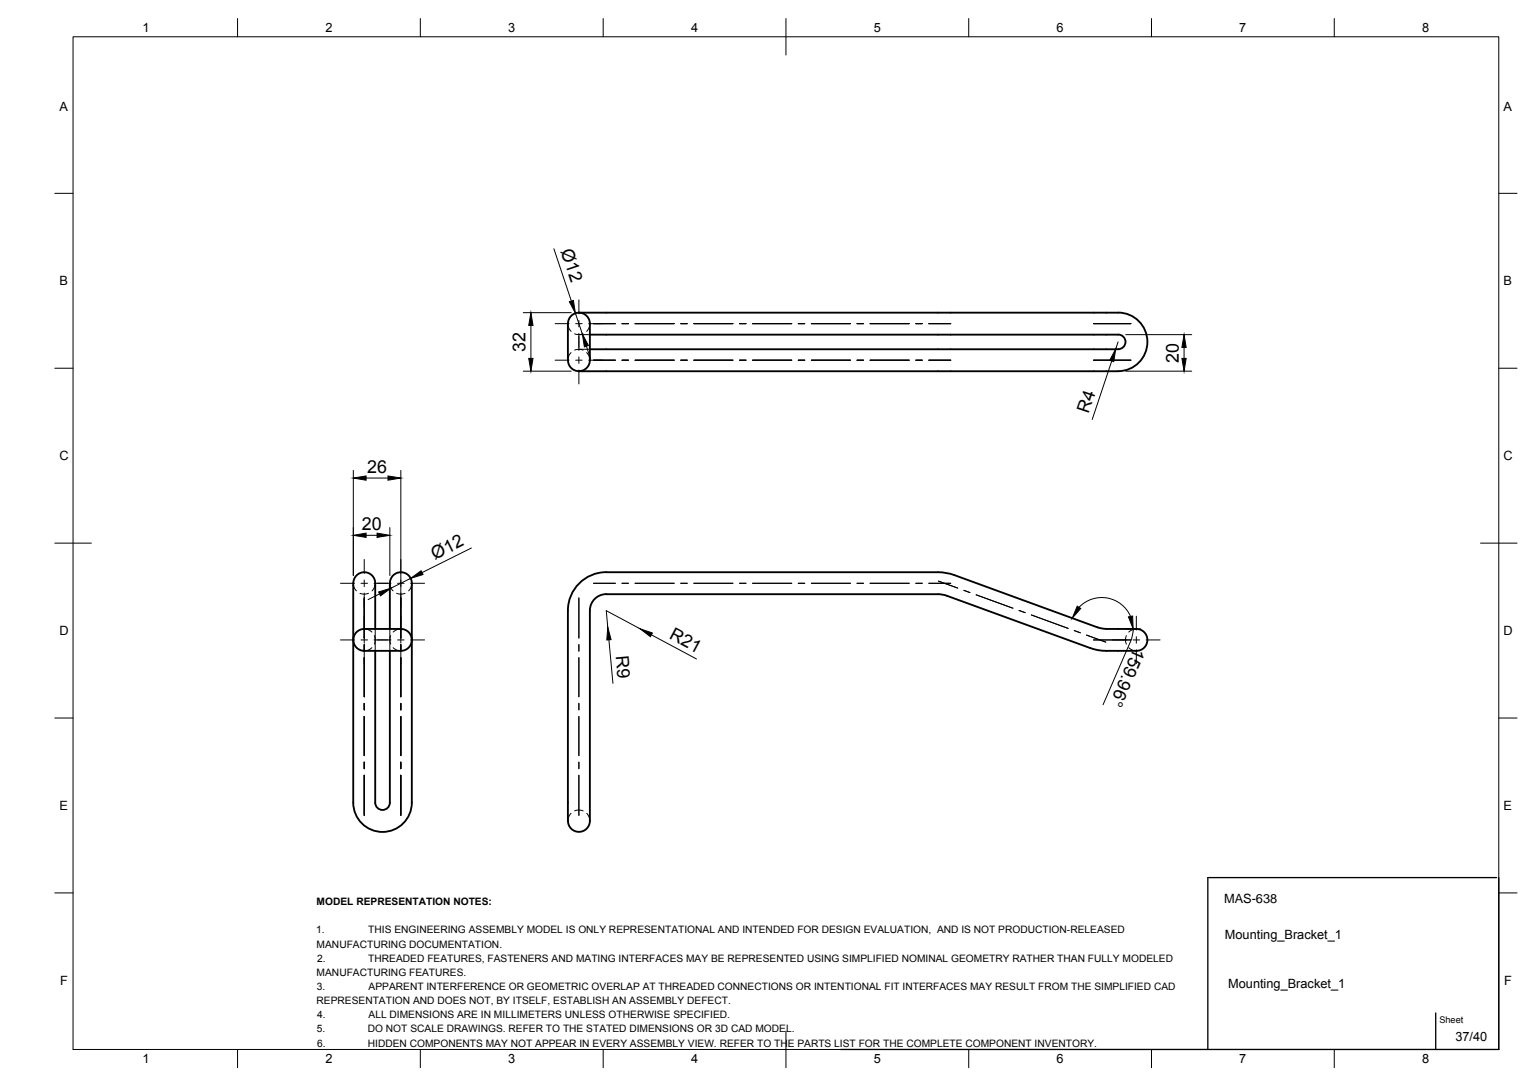
ISO-10303-21;
HEADER;
FILE_DESCRIPTION((''),'2;1');
FILE_NAME('Mounting_Bracket_1.step','2026-10-09T12:00:21-07:00',(''),(''),'','','');
FILE_SCHEMA (('AUTOMOTIVE_DESIGN { 1 0 10303 214 3 1 1 }'));
ENDSEC;
DATA;
#10=MECHANICAL_DESIGN_GEOMETRIC_PRESENTATION_REPRESENTATION('',(#432),#10334);
#160=CYLINDRICAL_SURFACE('',#4275,0.600000000000001) ;
#161=CYLINDRICAL_SURFACE('',#4276,0.600000000000001) ;
#162=CYLINDRICAL_SURFACE('',#4277,0.599999999999996) ;
#163=CYLINDRICAL_SURFACE('',#4278,0.600000000000001) ;
#164=CYLINDRICAL_SURFACE('',#4279,0.600000000000001) ;
#165=CYLINDRICAL_SURFACE('',#4280,0.600000000000001) ;
#166=CYLINDRICAL_SURFACE('',#4281,0.599999999999996) ;
#167=CYLINDRICAL_SURFACE('',#4282,0.600000000000001) ;
#360=SHAPE_REPRESENTATION_RELATIONSHIP('SRR','None',#10478,#392) ;
#392=ADVANCED_BREP_SHAPE_REPRESENTATION('',(#464),#10330) ;
#432=STYLED_ITEM('',(#10631),#464) ;
#464=MANIFOLD_SOLID_BREP('Body1',#3586) ;
#658=LINE('',#9983,#816) ;
#659=LINE('',#9985,#817) ;
#660=LINE('',#9987,#818) ;
#661=LINE('',#9989,#819) ;
#662=LINE('',#9991,#820) ;
#663=LINE('',#9993,#821) ;
#664=LINE('',#9995,#822) ;
#665=LINE('',#9997,#823) ;
#816=VECTOR('',#5236,0.600000000000001) ;
#817=VECTOR('',#5239,0.600000000000001) ;
#818=VECTOR('',#5242,0.599999999999996) ;
#819=VECTOR('',#5245,0.600000000000001) ;
#820=VECTOR('',#5248,0.600000000000001) ;
#821=VECTOR('',#5251,0.600000000000001) ;
#822=VECTOR('',#5254,0.599999999999996) ;
#823=VECTOR('',#5257,0.600000000000001) ;
#986=FACE_OUTER_BOUND('',#1194,.T.) ;
#987=FACE_OUTER_BOUND('',#1195,.T.) ;
#988=FACE_OUTER_BOUND('',#1196,.T.) ;
#989=FACE_OUTER_BOUND('',#1197,.T.) ;
#990=FACE_OUTER_BOUND('',#1198,.T.) ;
#991=FACE_OUTER_BOUND('',#1199,.T.) ;
#992=FACE_OUTER_BOUND('',#1200,.T.) ;
#993=FACE_OUTER_BOUND('',#1201,.T.) ;
#994=FACE_OUTER_BOUND('',#1202,.T.) ;
#995=FACE_OUTER_BOUND('',#1203,.T.) ;
#996=FACE_OUTER_BOUND('',#1204,.T.) ;
#997=FACE_OUTER_BOUND('',#1205,.T.) ;
#998=FACE_OUTER_BOUND('',#1206,.T.) ;
#999=FACE_OUTER_BOUND('',#1207,.T.) ;
#1000=FACE_OUTER_BOUND('',#1208,.T.) ;
#1001=FACE_OUTER_BOUND('',#1209,.T.) ;
#1194=EDGE_LOOP('',(#2965,#2966,#2967,#2968,#2969)) ;
#1195=EDGE_LOOP('',(#2970,#2971,#2972,#2973)) ;
#1196=EDGE_LOOP('',(#2974,#2975,#2976,#2977,#2978,#2979)) ;
#1197=EDGE_LOOP('',(#2980,#2981,#2982,#2983,#2984,#2985)) ;
#1198=EDGE_LOOP('',(#2986,#2987,#2988,#2989,#2990,#2991)) ;
#1199=EDGE_LOOP('',(#2992,#2993,#2994,#2995,#2996)) ;
#1200=EDGE_LOOP('',(#2997,#2998,#2999,#3000)) ;
#1201=EDGE_LOOP('',(#3001,#3002,#3003,#3004,#3005,#3006)) ;
#1202=EDGE_LOOP('',(#3007,#3008,#3009,#3010,#3011,#3012)) ;
#1203=EDGE_LOOP('',(#3013,#3014,#3015,#3016)) ;
#1204=EDGE_LOOP('',(#3017,#3018,#3019,#3020,#3021)) ;
#1205=EDGE_LOOP('',(#3022,#3023,#3024,#3025,#3026,#3027)) ;
#1206=EDGE_LOOP('',(#3028,#3029,#3030,#3031,#3032,#3033)) ;
#1207=EDGE_LOOP('',(#3034,#3035,#3036,#3037)) ;
#1208=EDGE_LOOP('',(#3038,#3039,#3040,#3041,#3042)) ;
#1209=EDGE_LOOP('',(#3043,#3044,#3045,#3046,#3047,#3048)) ;
#1363=CIRCLE('',#4234,0.600000000000001) ;
#1364=CIRCLE('',#4235,0.899999999999999) ;
#1365=CIRCLE('',#4236,0.600000000000001) ;
#1366=CIRCLE('',#4237,0.600000000000001) ;
#1367=CIRCLE('',#4239,0.600000000000001) ;
#1368=CIRCLE('',#4240,1.4) ;
#1369=CIRCLE('',#4241,0.600000000000001) ;
#1370=CIRCLE('',#4243,0.600000000000001) ;
#1371=CIRCLE('',#4244,0.600000000000001) ;
#1372=CIRCLE('',#4245,1.4) ;
#1373=CIRCLE('',#4246,0.600000000000001) ;
#1374=CIRCLE('',#4247,0.600000000000001) ;
#1375=CIRCLE('',#4249,0.600000000000001) ;
#1376=CIRCLE('',#4250,0.400000000000006) ;
#1377=CIRCLE('',#4251,0.600000000000001) ;
#1378=CIRCLE('',#4252,0.600000000000001) ;
#1379=CIRCLE('',#4253,0.600000000000001) ;
#1380=CIRCLE('',#4255,0.600000000000001) ;
#1381=CIRCLE('',#4256,0.600000000000001) ;
#1382=CIRCLE('',#4257,0.400000000000006) ;
#1383=CIRCLE('',#4258,0.600000000000001) ;
#1384=CIRCLE('',#4259,0.600000000000001) ;
#1385=CIRCLE('',#4261,0.600000000000001) ;
#1386=CIRCLE('',#4262,0.600000000000001) ;
#1387=CIRCLE('',#4263,0.899999999999999) ;
#1388=CIRCLE('',#4264,0.600000000000001) ;
#1389=CIRCLE('',#4266,0.600000000000001) ;
#1390=CIRCLE('',#4267,1.4) ;
#1391=CIRCLE('',#4268,0.600000000000001) ;
#1392=CIRCLE('',#4270,0.600000000000001) ;
#1393=CIRCLE('',#4271,0.600000000000001) ;
#1394=CIRCLE('',#4272,1.4) ;
#1395=CIRCLE('',#4273,0.600000000000001) ;
#1396=CIRCLE('',#4274,0.600000000000001) ;
#1706=VERTEX_POINT('',#9915) ;
#1707=VERTEX_POINT('',#9917) ;
#1708=VERTEX_POINT('',#9919) ;
#1709=VERTEX_POINT('',#9923) ;
#1710=VERTEX_POINT('',#9925) ;
#1711=VERTEX_POINT('',#9929) ;
#1712=VERTEX_POINT('',#9930) ;
#1713=VERTEX_POINT('',#9933) ;
#1714=VERTEX_POINT('',#9935) ;
#1715=VERTEX_POINT('',#9939) ;
#1716=VERTEX_POINT('',#9940) ;
#1717=VERTEX_POINT('',#9942) ;
#1718=VERTEX_POINT('',#9944) ;
#1719=VERTEX_POINT('',#9949) ;
#1720=VERTEX_POINT('',#9950) ;
#1721=VERTEX_POINT('',#9953) ;
#1722=VERTEX_POINT('',#9955) ;
#1723=VERTEX_POINT('',#9959) ;
#1724=VERTEX_POINT('',#9960) ;
#1725=VERTEX_POINT('',#9963) ;
#1726=VERTEX_POINT('',#9967) ;
#1727=VERTEX_POINT('',#9969) ;
#1728=VERTEX_POINT('',#9973) ;
#1729=VERTEX_POINT('',#9974) ;
#1730=VERTEX_POINT('',#9977) ;
#1731=VERTEX_POINT('',#9979) ;
#2139=EDGE_CURVE('',#1706,#1706,#1363,.T.) ;
#2140=EDGE_CURVE('',#1706,#1707,#1364,.T.) ;
#2141=EDGE_CURVE('',#1707,#1708,#1365,.T.) ;
#2142=EDGE_CURVE('',#1708,#1707,#1366,.T.) ;
#2143=EDGE_CURVE('',#1709,#1709,#1367,.T.) ;
#2144=EDGE_CURVE('',#1709,#1710,#1368,.T.) ;
#2145=EDGE_CURVE('',#1710,#1710,#1369,.T.) ;
#2146=EDGE_CURVE('',#1711,#1712,#1370,.T.) ;
#2147=EDGE_CURVE('',#1712,#1711,#1371,.T.) ;
#2148=EDGE_CURVE('',#1712,#1713,#1372,.T.) ;
#2149=EDGE_CURVE('',#1713,#1714,#1373,.T.) ;
#2150=EDGE_CURVE('',#1714,#1713,#1374,.T.) ;
#2151=EDGE_CURVE('',#1715,#1716,#1375,.T.) ;
#2152=EDGE_CURVE('',#1716,#1717,#1376,.T.) ;
#2153=EDGE_CURVE('',#1718,#1717,#1377,.T.) ;
#2154=EDGE_CURVE('',#1717,#1718,#1378,.T.) ;
#2155=EDGE_CURVE('',#1716,#1715,#1379,.T.) ;
#2156=EDGE_CURVE('',#1719,#1720,#1380,.T.) ;
#2157=EDGE_CURVE('',#1720,#1719,#1381,.T.) ;
#2158=EDGE_CURVE('',#1720,#1721,#1382,.T.) ;
#2159=EDGE_CURVE('',#1721,#1722,#1383,.T.) ;
#2160=EDGE_CURVE('',#1722,#1721,#1384,.T.) ;
#2161=EDGE_CURVE('',#1723,#1724,#1385,.T.) ;
#2162=EDGE_CURVE('',#1724,#1723,#1386,.T.) ;
#2163=EDGE_CURVE('',#1724,#1725,#1387,.T.) ;
#2164=EDGE_CURVE('',#1725,#1725,#1388,.T.) ;
#2165=EDGE_CURVE('',#1726,#1726,#1389,.T.) ;
#2166=EDGE_CURVE('',#1726,#1727,#1390,.T.) ;
#2167=EDGE_CURVE('',#1727,#1727,#1391,.T.) ;
#2168=EDGE_CURVE('',#1728,#1729,#1392,.T.) ;
#2169=EDGE_CURVE('',#1729,#1728,#1393,.T.) ;
#2170=EDGE_CURVE('',#1729,#1730,#1394,.T.) ;
#2171=EDGE_CURVE('',#1730,#1731,#1395,.T.) ;
#2172=EDGE_CURVE('',#1731,#1730,#1396,.T.) ;
#2173=EDGE_CURVE('',#1719,#1708,#658,.T.) ;
#2174=EDGE_CURVE('',#1706,#1710,#659,.T.) ;
#2175=EDGE_CURVE('',#1709,#1714,#660,.T.) ;
#2176=EDGE_CURVE('',#1711,#1715,#661,.T.) ;
#2177=EDGE_CURVE('',#1722,#1723,#662,.T.) ;
#2178=EDGE_CURVE('',#1725,#1726,#663,.T.) ;
#2179=EDGE_CURVE('',#1727,#1728,#664,.T.) ;
#2180=EDGE_CURVE('',#1731,#1718,#665,.T.) ;
#2965=ORIENTED_EDGE('',*,*,#2139,.F.) ;
#2966=ORIENTED_EDGE('',*,*,#2140,.T.) ;
#2967=ORIENTED_EDGE('',*,*,#2141,.T.) ;
#2968=ORIENTED_EDGE('',*,*,#2142,.T.) ;
#2969=ORIENTED_EDGE('',*,*,#2140,.F.) ;
#2970=ORIENTED_EDGE('',*,*,#2143,.F.) ;
#2971=ORIENTED_EDGE('',*,*,#2144,.T.) ;
#2972=ORIENTED_EDGE('',*,*,#2145,.T.) ;
#2973=ORIENTED_EDGE('',*,*,#2144,.F.) ;
#2974=ORIENTED_EDGE('',*,*,#2146,.F.) ;
#2975=ORIENTED_EDGE('',*,*,#2147,.F.) ;
#2976=ORIENTED_EDGE('',*,*,#2148,.T.) ;
#2977=ORIENTED_EDGE('',*,*,#2149,.T.) ;
#2978=ORIENTED_EDGE('',*,*,#2150,.T.) ;
#2979=ORIENTED_EDGE('',*,*,#2148,.F.) ;
#2980=ORIENTED_EDGE('',*,*,#2151,.T.) ;
#2981=ORIENTED_EDGE('',*,*,#2152,.T.) ;
#2982=ORIENTED_EDGE('',*,*,#2153,.F.) ;
#2983=ORIENTED_EDGE('',*,*,#2154,.F.) ;
#2984=ORIENTED_EDGE('',*,*,#2152,.F.) ;
#2985=ORIENTED_EDGE('',*,*,#2155,.T.) ;
#2986=ORIENTED_EDGE('',*,*,#2156,.F.) ;
#2987=ORIENTED_EDGE('',*,*,#2157,.F.) ;
#2988=ORIENTED_EDGE('',*,*,#2158,.T.) ;
#2989=ORIENTED_EDGE('',*,*,#2159,.T.) ;
#2990=ORIENTED_EDGE('',*,*,#2160,.T.) ;
#2991=ORIENTED_EDGE('',*,*,#2158,.F.) ;
#2992=ORIENTED_EDGE('',*,*,#2161,.F.) ;
#2993=ORIENTED_EDGE('',*,*,#2162,.F.) ;
#2994=ORIENTED_EDGE('',*,*,#2163,.T.) ;
#2995=ORIENTED_EDGE('',*,*,#2164,.T.) ;
#2996=ORIENTED_EDGE('',*,*,#2163,.F.) ;
#2997=ORIENTED_EDGE('',*,*,#2165,.F.) ;
#2998=ORIENTED_EDGE('',*,*,#2166,.T.) ;
#2999=ORIENTED_EDGE('',*,*,#2167,.T.) ;
#3000=ORIENTED_EDGE('',*,*,#2166,.F.) ;
#3001=ORIENTED_EDGE('',*,*,#2168,.F.) ;
#3002=ORIENTED_EDGE('',*,*,#2169,.F.) ;
#3003=ORIENTED_EDGE('',*,*,#2170,.T.) ;
#3004=ORIENTED_EDGE('',*,*,#2171,.T.) ;
#3005=ORIENTED_EDGE('',*,*,#2172,.T.) ;
#3006=ORIENTED_EDGE('',*,*,#2170,.F.) ;
#3007=ORIENTED_EDGE('',*,*,#2156,.T.) ;
#3008=ORIENTED_EDGE('',*,*,#2157,.T.) ;
#3009=ORIENTED_EDGE('',*,*,#2173,.T.) ;
#3010=ORIENTED_EDGE('',*,*,#2141,.F.) ;
#3011=ORIENTED_EDGE('',*,*,#2142,.F.) ;
#3012=ORIENTED_EDGE('',*,*,#2173,.F.) ;
#3013=ORIENTED_EDGE('',*,*,#2139,.T.) ;
#3014=ORIENTED_EDGE('',*,*,#2174,.T.) ;
#3015=ORIENTED_EDGE('',*,*,#2145,.F.) ;
#3016=ORIENTED_EDGE('',*,*,#2174,.F.) ;
#3017=ORIENTED_EDGE('',*,*,#2143,.T.) ;
#3018=ORIENTED_EDGE('',*,*,#2175,.T.) ;
#3019=ORIENTED_EDGE('',*,*,#2149,.F.) ;
#3020=ORIENTED_EDGE('',*,*,#2150,.F.) ;
#3021=ORIENTED_EDGE('',*,*,#2175,.F.) ;
#3022=ORIENTED_EDGE('',*,*,#2146,.T.) ;
#3023=ORIENTED_EDGE('',*,*,#2147,.T.) ;
#3024=ORIENTED_EDGE('',*,*,#2176,.T.) ;
#3025=ORIENTED_EDGE('',*,*,#2155,.F.) ;
#3026=ORIENTED_EDGE('',*,*,#2151,.F.) ;
#3027=ORIENTED_EDGE('',*,*,#2176,.F.) ;
#3028=ORIENTED_EDGE('',*,*,#2160,.F.) ;
#3029=ORIENTED_EDGE('',*,*,#2177,.T.) ;
#3030=ORIENTED_EDGE('',*,*,#2161,.T.) ;
#3031=ORIENTED_EDGE('',*,*,#2162,.T.) ;
#3032=ORIENTED_EDGE('',*,*,#2177,.F.) ;
#3033=ORIENTED_EDGE('',*,*,#2159,.F.) ;
#3034=ORIENTED_EDGE('',*,*,#2164,.F.) ;
#3035=ORIENTED_EDGE('',*,*,#2178,.T.) ;
#3036=ORIENTED_EDGE('',*,*,#2165,.T.) ;
#3037=ORIENTED_EDGE('',*,*,#2178,.F.) ;
#3038=ORIENTED_EDGE('',*,*,#2167,.F.) ;
#3039=ORIENTED_EDGE('',*,*,#2179,.T.) ;
#3040=ORIENTED_EDGE('',*,*,#2168,.T.) ;
#3041=ORIENTED_EDGE('',*,*,#2169,.T.) ;
#3042=ORIENTED_EDGE('',*,*,#2179,.F.) ;
#3043=ORIENTED_EDGE('',*,*,#2172,.F.) ;
#3044=ORIENTED_EDGE('',*,*,#2180,.T.) ;
#3045=ORIENTED_EDGE('',*,*,#2153,.T.) ;
#3046=ORIENTED_EDGE('',*,*,#2154,.T.) ;
#3047=ORIENTED_EDGE('',*,*,#2180,.F.) ;
#3048=ORIENTED_EDGE('',*,*,#2171,.F.) ;
#3327=TOROIDAL_SURFACE('',#4233,1.5,0.6) ;
#3328=TOROIDAL_SURFACE('',#4238,2.,0.6) ;
#3329=TOROIDAL_SURFACE('',#4242,2.,0.6) ;
#3330=TOROIDAL_SURFACE('',#4248,1.,0.6) ;
#3331=TOROIDAL_SURFACE('',#4254,1.,0.599999999999999) ;
#3332=TOROIDAL_SURFACE('',#4260,1.5,0.6) ;
#3333=TOROIDAL_SURFACE('',#4265,2.,0.6) ;
#3334=TOROIDAL_SURFACE('',#4269,2.,0.6) ;
#3494=ADVANCED_FACE('',(#986),#3327,.T.) ;
#3495=ADVANCED_FACE('',(#987),#3328,.T.) ;
#3496=ADVANCED_FACE('',(#988),#3329,.T.) ;
#3497=ADVANCED_FACE('',(#989),#3330,.T.) ;
#3498=ADVANCED_FACE('',(#990),#3331,.T.) ;
#3499=ADVANCED_FACE('',(#991),#3332,.T.) ;
#3500=ADVANCED_FACE('',(#992),#3333,.T.) ;
#3501=ADVANCED_FACE('',(#993),#3334,.T.) ;
#3502=ADVANCED_FACE('',(#994),#160,.T.) ;
#3503=ADVANCED_FACE('',(#995),#161,.T.) ;
#3504=ADVANCED_FACE('',(#996),#162,.T.) ;
#3505=ADVANCED_FACE('',(#997),#163,.T.) ;
#3506=ADVANCED_FACE('',(#998),#164,.T.) ;
#3507=ADVANCED_FACE('',(#999),#165,.T.) ;
#3508=ADVANCED_FACE('',(#1000),#166,.T.) ;
#3509=ADVANCED_FACE('',(#1001),#167,.T.) ;
#3586=CLOSED_SHELL('',(#3494,#3495,#3496,#3497,#3498,#3499,#3500,#3501,
#3502,#3503,#3504,#3505,#3506,#3507,#3508,#3509)) ;
#4232=AXIS2_PLACEMENT_3D('',#9913,#5148,#5149) ;
#4233=AXIS2_PLACEMENT_3D('',#9914,#5150,#5151) ;
#4234=AXIS2_PLACEMENT_3D('',#9916,#5152,#5153) ;
#4235=AXIS2_PLACEMENT_3D('',#9918,#5154,#5155) ;
#4236=AXIS2_PLACEMENT_3D('',#9920,#5156,#5157) ;
#4237=AXIS2_PLACEMENT_3D('',#9921,#5158,#5159) ;
#4238=AXIS2_PLACEMENT_3D('',#9922,#5160,#5161) ;
#4239=AXIS2_PLACEMENT_3D('',#9924,#5162,#5163) ;
#4240=AXIS2_PLACEMENT_3D('',#9926,#5164,#5165) ;
#4241=AXIS2_PLACEMENT_3D('',#9927,#5166,#5167) ;
#4242=AXIS2_PLACEMENT_3D('',#9928,#5168,#5169) ;
#4243=AXIS2_PLACEMENT_3D('',#9931,#5170,#5171) ;
#4244=AXIS2_PLACEMENT_3D('',#9932,#5172,#5173) ;
#4245=AXIS2_PLACEMENT_3D('',#9934,#5174,#5175) ;
#4246=AXIS2_PLACEMENT_3D('',#9936,#5176,#5177) ;
#4247=AXIS2_PLACEMENT_3D('',#9937,#5178,#5179) ;
#4248=AXIS2_PLACEMENT_3D('',#9938,#5180,#5181) ;
#4249=AXIS2_PLACEMENT_3D('',#9941,#5182,#5183) ;
#4250=AXIS2_PLACEMENT_3D('',#9943,#5184,#5185) ;
#4251=AXIS2_PLACEMENT_3D('',#9945,#5186,#5187) ;
#4252=AXIS2_PLACEMENT_3D('',#9946,#5188,#5189) ;
#4253=AXIS2_PLACEMENT_3D('',#9947,#5190,#5191) ;
#4254=AXIS2_PLACEMENT_3D('',#9948,#5192,#5193) ;
#4255=AXIS2_PLACEMENT_3D('',#9951,#5194,#5195) ;
#4256=AXIS2_PLACEMENT_3D('',#9952,#5196,#5197) ;
#4257=AXIS2_PLACEMENT_3D('',#9954,#5198,#5199) ;
#4258=AXIS2_PLACEMENT_3D('',#9956,#5200,#5201) ;
#4259=AXIS2_PLACEMENT_3D('',#9957,#5202,#5203) ;
#4260=AXIS2_PLACEMENT_3D('',#9958,#5204,#5205) ;
#4261=AXIS2_PLACEMENT_3D('',#9961,#5206,#5207) ;
#4262=AXIS2_PLACEMENT_3D('',#9962,#5208,#5209) ;
#4263=AXIS2_PLACEMENT_3D('',#9964,#5210,#5211) ;
#4264=AXIS2_PLACEMENT_3D('',#9965,#5212,#5213) ;
#4265=AXIS2_PLACEMENT_3D('',#9966,#5214,#5215) ;
#4266=AXIS2_PLACEMENT_3D('',#9968,#5216,#5217) ;
#4267=AXIS2_PLACEMENT_3D('',#9970,#5218,#5219) ;
#4268=AXIS2_PLACEMENT_3D('',#9971,#5220,#5221) ;
#4269=AXIS2_PLACEMENT_3D('',#9972,#5222,#5223) ;
#4270=AXIS2_PLACEMENT_3D('',#9975,#5224,#5225) ;
#4271=AXIS2_PLACEMENT_3D('',#9976,#5226,#5227) ;
#4272=AXIS2_PLACEMENT_3D('',#9978,#5228,#5229) ;
#4273=AXIS2_PLACEMENT_3D('',#9980,#5230,#5231) ;
#4274=AXIS2_PLACEMENT_3D('',#9981,#5232,#5233) ;
#4275=AXIS2_PLACEMENT_3D('',#9982,#5234,#5235) ;
#4276=AXIS2_PLACEMENT_3D('',#9984,#5237,#5238) ;
#4277=AXIS2_PLACEMENT_3D('',#9986,#5240,#5241) ;
#4278=AXIS2_PLACEMENT_3D('',#9988,#5243,#5244) ;
#4279=AXIS2_PLACEMENT_3D('',#9990,#5246,#5247) ;
#4280=AXIS2_PLACEMENT_3D('',#9992,#5249,#5250) ;
#4281=AXIS2_PLACEMENT_3D('',#9994,#5252,#5253) ;
#4282=AXIS2_PLACEMENT_3D('',#9996,#5255,#5256) ;
#5148=DIRECTION('axis',(0.,0.,1.)) ;
#5149=DIRECTION('refdir',(1.,0.,0.)) ;
#5150=DIRECTION('center_axis',(1.02015335365891E-16,0.,1.)) ;
#5151=DIRECTION('ref_axis',(-1.,0.,0.)) ;
#5152=DIRECTION('center_axis',(-1.,0.,1.02015335365891E-16)) ;
#5153=DIRECTION('ref_axis',(1.02015335365891E-16,0.,1.)) ;
#5154=DIRECTION('center_axis',(-1.02015335365891E-16,0.,-1.)) ;
#5155=DIRECTION('ref_axis',(-1.,0.,1.02015335365891E-16)) ;
#5156=DIRECTION('center_axis',(0.,1.,0.)) ;
#5157=DIRECTION('ref_axis',(0.,0.,1.)) ;
#5158=DIRECTION('center_axis',(0.,1.,0.)) ;
#5159=DIRECTION('ref_axis',(0.,0.,1.)) ;
#5160=DIRECTION('center_axis',(1.02015335365891E-16,0.,1.)) ;
#5161=DIRECTION('ref_axis',(-1.,0.,0.)) ;
#5162=DIRECTION('center_axis',(-0.93947030108257,-0.342630345100702,9.58403778312327E-17)) ;
#5163=DIRECTION('ref_axis',(9.00391886169754E-17,3.28378217308969E-17,1.)) ;
#5164=DIRECTION('center_axis',(-1.02015335365891E-16,0.,-1.)) ;
#5165=DIRECTION('ref_axis',(-1.,0.,1.02015335365891E-16)) ;
#5166=DIRECTION('center_axis',(-1.,0.,1.02015335365891E-16)) ;
#5167=DIRECTION('ref_axis',(1.02015335365891E-16,0.,1.)) ;
#5168=DIRECTION('center_axis',(-1.02015335365891E-16,0.,-1.)) ;
#5169=DIRECTION('ref_axis',(1.,0.,0.)) ;
#5170=DIRECTION('center_axis',(-1.,0.,1.02015335365891E-16)) ;
#5171=DIRECTION('ref_axis',(1.02015335365891E-16,0.,1.)) ;
#5172=DIRECTION('center_axis',(-1.,0.,1.02015335365891E-16)) ;
#5173=DIRECTION('ref_axis',(1.02015335365891E-16,0.,1.)) ;
#5174=DIRECTION('center_axis',(1.02015335365891E-16,0.,1.)) ;
#5175=DIRECTION('ref_axis',(1.,0.,-1.02015335365891E-16)) ;
#5176=DIRECTION('center_axis',(-0.93947030108257,-0.342630345100702,9.58403778312327E-17)) ;
#5177=DIRECTION('ref_axis',(9.00391886169754E-17,3.28378217308969E-17,1.)) ;
#5178=DIRECTION('center_axis',(-0.93947030108257,-0.342630345100702,9.58403778312327E-17)) ;
#5179=DIRECTION('ref_axis',(9.00391886169754E-17,3.28378217308969E-17,1.)) ;
#5180=DIRECTION('center_axis',(0.,-1.,0.)) ;
#5181=DIRECTION('ref_axis',(0.,0.,-1.)) ;
#5182=DIRECTION('center_axis',(-1.,0.,1.02015335365891E-16)) ;
#5183=DIRECTION('ref_axis',(1.02015335365891E-16,0.,1.)) ;
#5184=DIRECTION('center_axis',(0.,1.,0.)) ;
#5185=DIRECTION('ref_axis',(0.,0.,-1.)) ;
#5186=DIRECTION('center_axis',(1.,0.,0.)) ;
#5187=DIRECTION('ref_axis',(0.,0.,-1.)) ;
#5188=DIRECTION('center_axis',(1.,0.,0.)) ;
#5189=DIRECTION('ref_axis',(0.,0.,-1.)) ;
#5190=DIRECTION('center_axis',(-1.,0.,1.02015335365891E-16)) ;
#5191=DIRECTION('ref_axis',(1.02015335365891E-16,0.,1.)) ;
#5192=DIRECTION('center_axis',(1.,0.,0.)) ;
#5193=DIRECTION('ref_axis',(0.,0.,-1.)) ;
#5194=DIRECTION('center_axis',(0.,1.,0.)) ;
#5195=DIRECTION('ref_axis',(0.,0.,1.)) ;
#5196=DIRECTION('center_axis',(0.,1.,0.)) ;
#5197=DIRECTION('ref_axis',(0.,0.,1.)) ;
#5198=DIRECTION('center_axis',(-1.,0.,0.)) ;
#5199=DIRECTION('ref_axis',(0.,0.,-1.)) ;
#5200=DIRECTION('center_axis',(0.,-1.,0.)) ;
#5201=DIRECTION('ref_axis',(0.,0.,-1.)) ;
#5202=DIRECTION('center_axis',(0.,-1.,0.)) ;
#5203=DIRECTION('ref_axis',(0.,0.,-1.)) ;
#5204=DIRECTION('center_axis',(0.,0.,-1.)) ;
#5205=DIRECTION('ref_axis',(-1.,0.,0.)) ;
#5206=DIRECTION('center_axis',(0.,-1.,0.)) ;
#5207=DIRECTION('ref_axis',(0.,0.,-1.)) ;
#5208=DIRECTION('center_axis',(0.,-1.,0.)) ;
#5209=DIRECTION('ref_axis',(0.,0.,-1.)) ;
#5210=DIRECTION('center_axis',(0.,0.,1.)) ;
#5211=DIRECTION('ref_axis',(-1.,0.,0.)) ;
#5212=DIRECTION('center_axis',(1.,0.,0.)) ;
#5213=DIRECTION('ref_axis',(0.,0.,-1.)) ;
#5214=DIRECTION('center_axis',(0.,0.,-1.)) ;
#5215=DIRECTION('ref_axis',(-1.,0.,0.)) ;
#5216=DIRECTION('center_axis',(1.,0.,0.)) ;
#5217=DIRECTION('ref_axis',(0.,0.,-1.)) ;
#5218=DIRECTION('center_axis',(0.,0.,1.)) ;
#5219=DIRECTION('ref_axis',(-1.,0.,0.)) ;
#5220=DIRECTION('center_axis',(0.93947030108257,0.342630345100702,0.)) ;
#5221=DIRECTION('ref_axis',(0.,0.,-1.)) ;
#5222=DIRECTION('center_axis',(0.,0.,1.)) ;
#5223=DIRECTION('ref_axis',(1.,0.,0.)) ;
#5224=DIRECTION('center_axis',(0.93947030108257,0.342630345100702,0.)) ;
#5225=DIRECTION('ref_axis',(0.,0.,-1.)) ;
#5226=DIRECTION('center_axis',(0.93947030108257,0.342630345100702,0.)) ;
#5227=DIRECTION('ref_axis',(0.,0.,-1.)) ;
#5228=DIRECTION('center_axis',(0.,0.,-1.)) ;
#5229=DIRECTION('ref_axis',(1.,0.,0.)) ;
#5230=DIRECTION('center_axis',(1.,0.,0.)) ;
#5231=DIRECTION('ref_axis',(0.,0.,-1.)) ;
#5232=DIRECTION('center_axis',(1.,0.,0.)) ;
#5233=DIRECTION('ref_axis',(0.,0.,-1.)) ;
#5234=DIRECTION('center_axis',(0.,-1.,0.)) ;
#5235=DIRECTION('ref_axis',(0.,0.,1.)) ;
#5236=DIRECTION('',(0.,1.,0.)) ;
#5237=DIRECTION('center_axis',(1.,1.91189112624469E-17,-1.02015335365891E-16)) ;
#5238=DIRECTION('ref_axis',(-1.91189112624469E-17,1.,1.95042214426922E-33)) ;
#5239=DIRECTION('',(-1.,-1.91189112624469E-17,1.02015335365891E-16)) ;
#5240=DIRECTION('center_axis',(0.93947030108257,0.342630345100702,-9.58403778312327E-17)) ;
#5241=DIRECTION('ref_axis',(-0.342630345100702,0.93947030108257,3.97141584069169E-32)) ;
#5242=DIRECTION('',(-0.93947030108257,-0.342630345100702,9.58403778312327E-17)) ;
#5243=DIRECTION('center_axis',(1.,0.,-1.02015335365891E-16)) ;
#5244=DIRECTION('ref_axis',(1.02015335365891E-16,0.,1.)) ;
#5245=DIRECTION('',(-1.,0.,1.02015335365891E-16)) ;
#5246=DIRECTION('center_axis',(0.,-1.,0.)) ;
#5247=DIRECTION('ref_axis',(0.,0.,-1.)) ;
#5248=DIRECTION('',(0.,1.,0.)) ;
#5249=DIRECTION('center_axis',(1.,1.91189112624469E-17,0.)) ;
#5250=DIRECTION('ref_axis',(-1.91189112624469E-17,1.,0.)) ;
#5251=DIRECTION('',(-1.,-1.91189112624469E-17,0.)) ;
#5252=DIRECTION('center_axis',(0.93947030108257,0.342630345100702,0.)) ;
#5253=DIRECTION('ref_axis',(-0.342630345100702,0.93947030108257,0.)) ;
#5254=DIRECTION('',(-0.93947030108257,-0.342630345100702,0.)) ;
#5255=DIRECTION('center_axis',(1.,0.,0.)) ;
#5256=DIRECTION('ref_axis',(0.,0.,-1.)) ;
#5257=DIRECTION('',(-1.,0.,0.)) ;
#9913=CARTESIAN_POINT('',(0.,0.,0.)) ;
#9914=CARTESIAN_POINT('Origin',(58.7276880157606,67.0830586252741,67.2224337400009)) ;
#9915=CARTESIAN_POINT('',(58.7276880157606,67.9830586252741,67.2224337400009)) ;
#9916=CARTESIAN_POINT('Origin',(58.7276880157606,68.5830586252741,67.2224337400009)) ;
#9917=CARTESIAN_POINT('',(59.6276880157606,67.0830586252741,67.2224337400009)) ;
#9918=CARTESIAN_POINT('Origin',(58.7276880157606,67.0830586252741,67.2224337400009)) ;
#9919=CARTESIAN_POINT('',(60.2276880157606,67.0830586252741,66.6224337400009)) ;
#9920=CARTESIAN_POINT('Origin',(60.2276880157606,67.0830586252741,67.2224337400009)) ;
#9921=CARTESIAN_POINT('Origin',(60.2276880157606,67.0830586252741,67.2224337400009)) ;
#9922=CARTESIAN_POINT('Origin',(40.5810116473826,66.5830586252741,67.2224337400009)) ;
#9923=CARTESIAN_POINT('',(40.1013291642416,67.8983170467897,67.2224337400009)) ;
#9924=CARTESIAN_POINT('Origin',(39.8957509571812,68.4619992274392,67.2224337400009)) ;
#9925=CARTESIAN_POINT('',(40.5810116473826,67.9830586252741,67.2224337400009)) ;
#9926=CARTESIAN_POINT('Origin',(40.5810116473826,66.5830586252741,67.2224337400009)) ;
#9927=CARTESIAN_POINT('Origin',(40.5810116473826,68.5830586252741,67.2224337400009)) ;
#9928=CARTESIAN_POINT('Origin',(31.3743643841387,67.4830586252741,67.2224337400009)) ;
#9929=CARTESIAN_POINT('',(31.3743643841387,65.4830586252741,66.6224337400009)) ;
#9930=CARTESIAN_POINT('',(31.3743643841387,66.0830586252741,67.2224337400009)) ;
#9931=CARTESIAN_POINT('Origin',(31.3743643841387,65.4830586252741,67.2224337400009)) ;
#9932=CARTESIAN_POINT('Origin',(31.3743643841387,65.4830586252741,67.2224337400009)) ;
#9933=CARTESIAN_POINT('',(31.8540468672797,66.1678002037585,67.2224337400009)) ;
#9934=CARTESIAN_POINT('Origin',(31.3743643841387,67.4830586252741,67.2224337400009)) ;
#9935=CARTESIAN_POINT('',(32.2652032814005,65.0404358424594,67.2224337400009)) ;
#9936=CARTESIAN_POINT('Origin',(32.0596250743401,65.604118023109,67.2224337400009)) ;
#9937=CARTESIAN_POINT('Origin',(32.0596250743401,65.604118023109,67.2224337400009)) ;
#9938=CARTESIAN_POINT('Origin',(30.7276880157606,65.4830586252741,68.2224337400009)) ;
#9939=CARTESIAN_POINT('',(30.7276880157606,65.4830586252741,66.6224337400009)) ;
#9940=CARTESIAN_POINT('',(30.7276880157606,65.4830586252741,67.8224337400009)) ;
#9941=CARTESIAN_POINT('Origin',(30.7276880157606,65.4830586252741,67.2224337400009)) ;
#9942=CARTESIAN_POINT('',(30.7276880157606,65.4830586252741,68.6224337400009)) ;
#9943=CARTESIAN_POINT('Origin',(30.7276880157606,65.4830586252741,68.2224337400009)) ;
#9944=CARTESIAN_POINT('',(30.7276880157606,65.4830586252741,69.8224337400008)) ;
#9945=CARTESIAN_POINT('Origin',(30.7276880157606,65.4830586252741,69.2224337400009)) ;
#9946=CARTESIAN_POINT('Origin',(30.7276880157606,65.4830586252741,69.2224337400009)) ;
#9947=CARTESIAN_POINT('Origin',(30.7276880157606,65.4830586252741,67.2224337400009)) ;
#9948=CARTESIAN_POINT('Origin',(60.2276880157606,56.5830586252741,68.2224337400009)) ;
#9949=CARTESIAN_POINT('',(60.2276880157606,56.5830586252741,66.6224337400009)) ;
#9950=CARTESIAN_POINT('',(60.2276880157606,56.5830586252741,67.8224337400009)) ;
#9951=CARTESIAN_POINT('Origin',(60.2276880157606,56.5830586252741,67.2224337400009)) ;
#9952=CARTESIAN_POINT('Origin',(60.2276880157606,56.5830586252741,67.2224337400009)) ;
#9953=CARTESIAN_POINT('',(60.2276880157606,56.5830586252741,68.6224337400009)) ;
#9954=CARTESIAN_POINT('Origin',(60.2276880157606,56.5830586252741,68.2224337400009)) ;
#9955=CARTESIAN_POINT('',(60.2276880157606,56.5830586252741,69.8224337400008)) ;
#9956=CARTESIAN_POINT('Origin',(60.2276880157606,56.5830586252741,69.2224337400009)) ;
#9957=CARTESIAN_POINT('Origin',(60.2276880157606,56.5830586252741,69.2224337400009)) ;
#9958=CARTESIAN_POINT('Origin',(58.7276880157606,67.0830586252741,69.2224337400009)) ;
#9959=CARTESIAN_POINT('',(60.2276880157606,67.0830586252741,69.8224337400008)) ;
#9960=CARTESIAN_POINT('',(59.6276880157606,67.0830586252741,69.2224337400009)) ;
#9961=CARTESIAN_POINT('Origin',(60.2276880157606,67.0830586252741,69.2224337400009)) ;
#9962=CARTESIAN_POINT('Origin',(60.2276880157606,67.0830586252741,69.2224337400009)) ;
#9963=CARTESIAN_POINT('',(58.7276880157606,67.9830586252741,69.2224337400009)) ;
#9964=CARTESIAN_POINT('Origin',(58.7276880157606,67.0830586252741,69.2224337400009)) ;
#9965=CARTESIAN_POINT('Origin',(58.7276880157606,68.5830586252741,69.2224337400009)) ;
#9966=CARTESIAN_POINT('Origin',(40.5810116473826,66.5830586252741,69.2224337400009)) ;
#9967=CARTESIAN_POINT('',(40.5810116473826,67.9830586252741,69.2224337400009)) ;
#9968=CARTESIAN_POINT('Origin',(40.5810116473826,68.5830586252741,69.2224337400009)) ;
#9969=CARTESIAN_POINT('',(40.1013291642416,67.8983170467897,69.2224337400009)) ;
#9970=CARTESIAN_POINT('Origin',(40.5810116473826,66.5830586252741,69.2224337400009)) ;
#9971=CARTESIAN_POINT('Origin',(39.8957509571812,68.4619992274392,69.2224337400009)) ;
#9972=CARTESIAN_POINT('Origin',(31.3743643841387,67.4830586252741,69.2224337400009)) ;
#9973=CARTESIAN_POINT('',(32.2652032814005,65.0404358424594,69.2224337400009)) ;
#9974=CARTESIAN_POINT('',(31.8540468672797,66.1678002037585,69.2224337400009)) ;
#9975=CARTESIAN_POINT('Origin',(32.0596250743401,65.604118023109,69.2224337400009)) ;
#9976=CARTESIAN_POINT('Origin',(32.0596250743401,65.604118023109,69.2224337400009)) ;
#9977=CARTESIAN_POINT('',(31.3743643841387,66.0830586252741,69.2224337400009)) ;
#9978=CARTESIAN_POINT('Origin',(31.3743643841387,67.4830586252741,69.2224337400009)) ;
#9979=CARTESIAN_POINT('',(31.3743643841387,65.4830586252741,69.8224337400008)) ;
#9980=CARTESIAN_POINT('Origin',(31.3743643841387,65.4830586252741,69.2224337400009)) ;
#9981=CARTESIAN_POINT('Origin',(31.3743643841387,65.4830586252741,69.2224337400009)) ;
#9982=CARTESIAN_POINT('Origin',(60.2276880157606,67.0830586252741,67.2224337400009)) ;
#9983=CARTESIAN_POINT('',(60.2276880157606,67.0830586252741,66.6224337400009)) ;
#9984=CARTESIAN_POINT('Origin',(40.5810116473826,68.5830586252741,67.2224337400009)) ;
#9985=CARTESIAN_POINT('',(40.5810116473826,67.9830586252741,67.2224337400009)) ;
#9986=CARTESIAN_POINT('Origin',(32.0596250743401,65.6041180231089,67.2224337400009)) ;
#9987=CARTESIAN_POINT('',(32.2652032814005,65.0404358424594,67.2224337400009)) ;
#9988=CARTESIAN_POINT('Origin',(30.7276880157606,65.4830586252741,67.2224337400009)) ;
#9989=CARTESIAN_POINT('',(30.7276880157606,65.4830586252741,66.6224337400009)) ;
#9990=CARTESIAN_POINT('Origin',(60.2276880157606,67.0830586252741,69.2224337400009)) ;
#9991=CARTESIAN_POINT('',(60.2276880157606,67.0830586252741,69.8224337400009)) ;
#9992=CARTESIAN_POINT('Origin',(40.5810116473826,68.5830586252741,69.2224337400009)) ;
#9993=CARTESIAN_POINT('',(40.5810116473826,67.9830586252741,69.2224337400009)) ;
#9994=CARTESIAN_POINT('Origin',(32.0596250743401,65.6041180231089,69.2224337400009)) ;
#9995=CARTESIAN_POINT('',(32.2652032814005,65.0404358424594,69.2224337400009)) ;
#9996=CARTESIAN_POINT('Origin',(30.7276880157606,65.4830586252741,69.2224337400009)) ;
#9997=CARTESIAN_POINT('',(30.7276880157606,65.4830586252741,69.8224337400009)) ;
#10293=UNCERTAINTY_MEASURE_WITH_UNIT(LENGTH_MEASURE(0.001),#10335,
'DISTANCE_ACCURACY_VALUE',
'Maximum model space distance between geometric entities at asserted c
onnectivities') ;
#10297=UNCERTAINTY_MEASURE_WITH_UNIT(LENGTH_MEASURE(0.001),#10335,
'DISTANCE_ACCURACY_VALUE',
'Maximum model space distance between geometric entities at asserted c
onnectivities') ;
#10330=(
GEOMETRIC_REPRESENTATION_CONTEXT(3)
GLOBAL_UNCERTAINTY_ASSIGNED_CONTEXT((#10293))
GLOBAL_UNIT_ASSIGNED_CONTEXT((#10335,#10337,#10338))
REPRESENTATION_CONTEXT('','3D')
) ;
#10334=(
GEOMETRIC_REPRESENTATION_CONTEXT(3)
GLOBAL_UNCERTAINTY_ASSIGNED_CONTEXT((#10297))
GLOBAL_UNIT_ASSIGNED_CONTEXT((#10335,#10337,#10338))
REPRESENTATION_CONTEXT('','3D')
) ;
#10335=(
LENGTH_UNIT()
NAMED_UNIT(*)
SI_UNIT(.CENTI.,.METRE.)
) ;
#10337=(
NAMED_UNIT(*)
PLANE_ANGLE_UNIT()
SI_UNIT($,.RADIAN.)
) ;
#10338=(
NAMED_UNIT(*)
SI_UNIT($,.STERADIAN.)
SOLID_ANGLE_UNIT()
) ;
#10371=SHAPE_DEFINITION_REPRESENTATION(#10434,#10478) ;
#10434=PRODUCT_DEFINITION_SHAPE('',$,#10515) ;
#10478=SHAPE_REPRESENTATION('',(#4232),#10330) ;
#10482=PRODUCT_DEFINITION_CONTEXT('part definition',#10592,'design') ;
#10515=PRODUCT_DEFINITION('Mounting_Bracket_1','Mounting_Bracket_1',#10551,
#10482) ;
#10551=PRODUCT_DEFINITION_FORMATION('',$,#10626) ;
#10592=APPLICATION_CONTEXT(
'Core Data for Automotive Mechanical Design Process') ;
#10593=PRODUCT_CONTEXT('part definition',#10592,'mechanical') ;
#10626=PRODUCT('Mounting_Bracket_1','Mounting_Bracket_1',$,(#10593)) ;
#10631=PRESENTATION_STYLE_ASSIGNMENT((#10635)) ;
#10635=SURFACE_STYLE_USAGE(.BOTH.,#10639) ;
#10639=SURFACE_SIDE_STYLE('',(#10643)) ;
#10643=SURFACE_STYLE_FILL_AREA(#10647) ;
#10647=FILL_AREA_STYLE('Opaque(25,25,25)',(#10651)) ;
#10651=FILL_AREA_STYLE_COLOUR('Opaque(25,25,25)',#10655) ;
#10655=COLOUR_RGB('Opaque(25,25,25)', 0.09019608, 0.27058824, 0.51372549) ;
ENDSEC;
END-ISO-10303-21;
